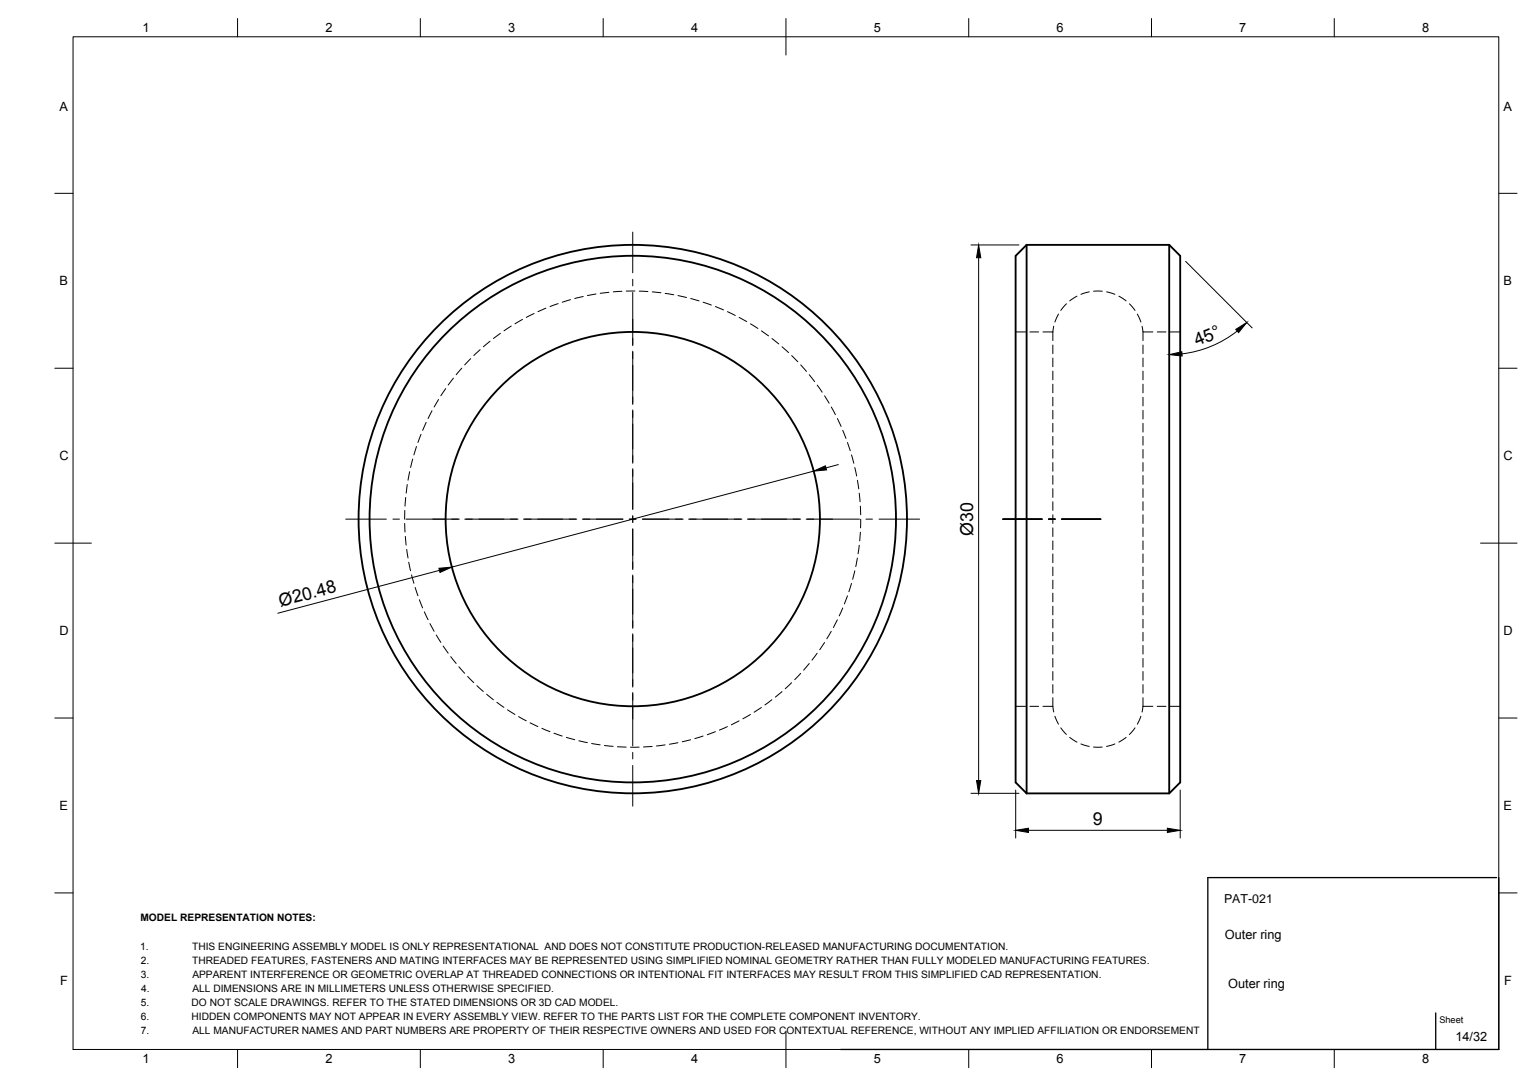
ISO-10303-21;
HEADER;
/* Generated by software containing ST-Developer
 * from STEP Tools, Inc. (www.steptools.com) 
 */

FILE_DESCRIPTION(
/* description */ ('Chain-less indexing wheel (Geneva) drive'),
/* implementation_level */ '2;1');

FILE_NAME(
/* name */ 'Outer ring.step',
/* time_stamp */ '2026-10-28T03:25:22-07:00',
/* author */ (''),
/* organization */ (''),
/* preprocessor_version */ 'ST-DEVELOPER v20.2',
/* originating_system */ 'Autodesk Translation Framework v15.17.0.0',
/* authorisation */ '');

FILE_SCHEMA (('AUTOMOTIVE_DESIGN { 1 0 10303 214 3 1 1 }'));
ENDSEC;

DATA;
#10=MECHANICAL_DESIGN_GEOMETRIC_PRESENTATION_REPRESENTATION('',(#311),#10957);
#196=TOROIDAL_SURFACE('',#6292,1.,0.247676);
#205=CONICAL_SURFACE('',#6303,1.47,0.785398163397449);
#206=CONICAL_SURFACE('',#6307,1.47,0.785398163397449);
#261=SHAPE_REPRESENTATION_RELATIONSHIP('SRR','None',#11075,#286);
#286=ADVANCED_BREP_SHAPE_REPRESENTATION('',(#343),#10938);
#311=STYLED_ITEM('',(#11287),#343);
#343=MANIFOLD_SOLID_BREP('Body1',#5708);
#426=FACE_BOUND('',#1180,.T.);
#427=FACE_BOUND('',#1185,.T.);
#541=PLANE('',#6300);
#542=PLANE('',#6309);
#785=FACE_OUTER_BOUND('',#1177,.T.);
#786=FACE_OUTER_BOUND('',#1178,.T.);
#787=FACE_OUTER_BOUND('',#1179,.T.);
#788=FACE_OUTER_BOUND('',#1181,.T.);
#789=FACE_OUTER_BOUND('',#1182,.T.);
#790=FACE_OUTER_BOUND('',#1183,.T.);
#791=FACE_OUTER_BOUND('',#1184,.T.);
#792=FACE_OUTER_BOUND('',#1186,.T.);
#1177=EDGE_LOOP('',(#4331,#4332,#4333,#4334,#4335,#4336));
#1178=EDGE_LOOP('',(#4337,#4338,#4339,#4340,#4341));
#1179=EDGE_LOOP('',(#4342));
#1180=EDGE_LOOP('',(#4343));
#1181=EDGE_LOOP('',(#4344,#4345,#4346,#4347));
#1182=EDGE_LOOP('',(#4348,#4349,#4350,#4351));
#1183=EDGE_LOOP('',(#4352,#4353,#4354,#4355));
#1184=EDGE_LOOP('',(#4356));
#1185=EDGE_LOOP('',(#4357));
#1186=EDGE_LOOP('',(#4358,#4359,#4360,#4361,#4362));
#1576=LINE('',#9299,#1950);
#1577=LINE('',#9308,#1951);
#1578=LINE('',#9312,#1952);
#1579=LINE('',#9316,#1953);
#1580=LINE('',#9319,#1954);
#1950=VECTOR('',#7482,1.023815);
#1951=VECTOR('',#7493,1.47);
#1952=VECTOR('',#7498,1.5);
#1953=VECTOR('',#7503,1.47);
#1954=VECTOR('',#7508,1.023815);
#2308=CIRCLE('',#6293,1.023815);
#2309=CIRCLE('',#6294,1.023815);
#2310=CIRCLE('',#6295,0.247676);
#2311=CIRCLE('',#6296,1.023815);
#2312=CIRCLE('',#6297,1.023815);
#2313=CIRCLE('',#6299,1.023815);
#2314=CIRCLE('',#6301,1.44);
#2315=CIRCLE('',#6302,1.023815);
#2316=CIRCLE('',#6304,1.5);
#2317=CIRCLE('',#6306,1.5);
#2318=CIRCLE('',#6308,1.44);
#2687=VERTEX_POINT('',#9287);
#2688=VERTEX_POINT('',#9288);
#2689=VERTEX_POINT('',#9291);
#2690=VERTEX_POINT('',#9293);
#2691=VERTEX_POINT('',#9297);
#2692=VERTEX_POINT('',#9301);
#2693=VERTEX_POINT('',#9303);
#2694=VERTEX_POINT('',#9306);
#2695=VERTEX_POINT('',#9310);
#2696=VERTEX_POINT('',#9314);
#3291=EDGE_CURVE('',#2687,#2688,#2308,.T.);
#3292=EDGE_CURVE('',#2688,#2687,#2309,.T.);
#3293=EDGE_CURVE('',#2688,#2689,#2310,.T.);
#3294=EDGE_CURVE('',#2690,#2689,#2311,.T.);
#3295=EDGE_CURVE('',#2689,#2690,#2312,.T.);
#3296=EDGE_CURVE('',#2691,#2691,#2313,.T.);
#3297=EDGE_CURVE('',#2691,#2690,#1576,.T.);
#3298=EDGE_CURVE('',#2692,#2692,#2314,.T.);
#3299=EDGE_CURVE('',#2693,#2693,#2315,.T.);
#3300=EDGE_CURVE('',#2694,#2694,#2316,.T.);
#3301=EDGE_CURVE('',#2694,#2692,#1577,.T.);
#3302=EDGE_CURVE('',#2695,#2695,#2317,.T.);
#3303=EDGE_CURVE('',#2695,#2694,#1578,.T.);
#3304=EDGE_CURVE('',#2696,#2696,#2318,.T.);
#3305=EDGE_CURVE('',#2696,#2695,#1579,.T.);
#3306=EDGE_CURVE('',#2687,#2693,#1580,.T.);
#4331=ORIENTED_EDGE('',*,*,#3291,.F.);
#4332=ORIENTED_EDGE('',*,*,#3292,.F.);
#4333=ORIENTED_EDGE('',*,*,#3293,.T.);
#4334=ORIENTED_EDGE('',*,*,#3294,.F.);
#4335=ORIENTED_EDGE('',*,*,#3295,.F.);
#4336=ORIENTED_EDGE('',*,*,#3293,.F.);
#4337=ORIENTED_EDGE('',*,*,#3296,.T.);
#4338=ORIENTED_EDGE('',*,*,#3297,.T.);
#4339=ORIENTED_EDGE('',*,*,#3294,.T.);
#4340=ORIENTED_EDGE('',*,*,#3295,.T.);
#4341=ORIENTED_EDGE('',*,*,#3297,.F.);
#4342=ORIENTED_EDGE('',*,*,#3298,.F.);
#4343=ORIENTED_EDGE('',*,*,#3299,.T.);
#4344=ORIENTED_EDGE('',*,*,#3300,.F.);
#4345=ORIENTED_EDGE('',*,*,#3301,.T.);
#4346=ORIENTED_EDGE('',*,*,#3298,.T.);
#4347=ORIENTED_EDGE('',*,*,#3301,.F.);
#4348=ORIENTED_EDGE('',*,*,#3302,.F.);
#4349=ORIENTED_EDGE('',*,*,#3303,.T.);
#4350=ORIENTED_EDGE('',*,*,#3300,.T.);
#4351=ORIENTED_EDGE('',*,*,#3303,.F.);
#4352=ORIENTED_EDGE('',*,*,#3304,.F.);
#4353=ORIENTED_EDGE('',*,*,#3305,.T.);
#4354=ORIENTED_EDGE('',*,*,#3302,.T.);
#4355=ORIENTED_EDGE('',*,*,#3305,.F.);
#4356=ORIENTED_EDGE('',*,*,#3304,.T.);
#4357=ORIENTED_EDGE('',*,*,#3296,.F.);
#4358=ORIENTED_EDGE('',*,*,#3291,.T.);
#4359=ORIENTED_EDGE('',*,*,#3292,.T.);
#4360=ORIENTED_EDGE('',*,*,#3306,.T.);
#4361=ORIENTED_EDGE('',*,*,#3299,.F.);
#4362=ORIENTED_EDGE('',*,*,#3306,.F.);
#5300=CYLINDRICAL_SURFACE('',#6298,1.023815);
#5301=CYLINDRICAL_SURFACE('',#6305,1.5);
#5302=CYLINDRICAL_SURFACE('',#6310,1.023815);
#5499=ADVANCED_FACE('',(#785),#196,.F.);
#5500=ADVANCED_FACE('',(#786),#5300,.F.);
#5501=ADVANCED_FACE('',(#787,#426),#541,.T.);
#5502=ADVANCED_FACE('',(#788),#205,.T.);
#5503=ADVANCED_FACE('',(#789),#5301,.T.);
#5504=ADVANCED_FACE('',(#790),#206,.T.);
#5505=ADVANCED_FACE('',(#791,#427),#542,.T.);
#5506=ADVANCED_FACE('',(#792),#5302,.F.);
#5708=CLOSED_SHELL('',(#5499,#5500,#5501,#5502,#5503,#5504,#5505,#5506));
#6291=AXIS2_PLACEMENT_3D('',#9285,#7464,#7465);
#6292=AXIS2_PLACEMENT_3D('',#9286,#7466,#7467);
#6293=AXIS2_PLACEMENT_3D('',#9289,#7468,#7469);
#6294=AXIS2_PLACEMENT_3D('',#9290,#7470,#7471);
#6295=AXIS2_PLACEMENT_3D('',#9292,#7472,#7473);
#6296=AXIS2_PLACEMENT_3D('',#9294,#7474,#7475);
#6297=AXIS2_PLACEMENT_3D('',#9295,#7476,#7477);
#6298=AXIS2_PLACEMENT_3D('',#9296,#7478,#7479);
#6299=AXIS2_PLACEMENT_3D('',#9298,#7480,#7481);
#6300=AXIS2_PLACEMENT_3D('',#9300,#7483,#7484);
#6301=AXIS2_PLACEMENT_3D('',#9302,#7485,#7486);
#6302=AXIS2_PLACEMENT_3D('',#9304,#7487,#7488);
#6303=AXIS2_PLACEMENT_3D('',#9305,#7489,#7490);
#6304=AXIS2_PLACEMENT_3D('',#9307,#7491,#7492);
#6305=AXIS2_PLACEMENT_3D('',#9309,#7494,#7495);
#6306=AXIS2_PLACEMENT_3D('',#9311,#7496,#7497);
#6307=AXIS2_PLACEMENT_3D('',#9313,#7499,#7500);
#6308=AXIS2_PLACEMENT_3D('',#9315,#7501,#7502);
#6309=AXIS2_PLACEMENT_3D('',#9317,#7504,#7505);
#6310=AXIS2_PLACEMENT_3D('',#9318,#7506,#7507);
#7464=DIRECTION('axis',(0.,0.,1.));
#7465=DIRECTION('refdir',(1.,0.,0.));
#7466=DIRECTION('center_axis',(0.,-1.,0.));
#7467=DIRECTION('ref_axis',(0.,0.,-1.));
#7468=DIRECTION('center_axis',(0.,-1.,0.));
#7469=DIRECTION('ref_axis',(1.,0.,0.));
#7470=DIRECTION('center_axis',(0.,-1.,0.));
#7471=DIRECTION('ref_axis',(1.,0.,0.));
#7472=DIRECTION('center_axis',(1.,0.,1.22464679914735E-16));
#7473=DIRECTION('ref_axis',(-1.22464679914735E-16,0.,1.));
#7474=DIRECTION('center_axis',(0.,1.,0.));
#7475=DIRECTION('ref_axis',(1.,0.,0.));
#7476=DIRECTION('center_axis',(0.,1.,0.));
#7477=DIRECTION('ref_axis',(1.,0.,0.));
#7478=DIRECTION('center_axis',(0.,-1.,0.));
#7479=DIRECTION('ref_axis',(1.,0.,0.));
#7480=DIRECTION('center_axis',(0.,-1.,0.));
#7481=DIRECTION('ref_axis',(1.,0.,0.));
#7482=DIRECTION('',(0.,1.,0.));
#7483=DIRECTION('center_axis',(0.,1.,0.));
#7484=DIRECTION('ref_axis',(0.,0.,1.));
#7485=DIRECTION('center_axis',(0.,-1.,0.));
#7486=DIRECTION('ref_axis',(1.,0.,0.));
#7487=DIRECTION('center_axis',(0.,-1.,0.));
#7488=DIRECTION('ref_axis',(1.,0.,0.));
#7489=DIRECTION('center_axis',(0.,-1.,0.));
#7490=DIRECTION('ref_axis',(1.,0.,0.));
#7491=DIRECTION('center_axis',(0.,-1.,0.));
#7492=DIRECTION('ref_axis',(1.,0.,0.));
#7493=DIRECTION('',(0.707106781186548,0.707106781186547,8.65956056235494E-17));
#7494=DIRECTION('center_axis',(0.,-1.,0.));
#7495=DIRECTION('ref_axis',(1.,0.,0.));
#7496=DIRECTION('center_axis',(0.,-1.,0.));
#7497=DIRECTION('ref_axis',(1.,0.,0.));
#7498=DIRECTION('',(0.,1.,0.));
#7499=DIRECTION('center_axis',(0.,1.,0.));
#7500=DIRECTION('ref_axis',(1.,0.,0.));
#7501=DIRECTION('center_axis',(0.,-1.,0.));
#7502=DIRECTION('ref_axis',(1.,0.,0.));
#7503=DIRECTION('',(-0.707106781186548,0.707106781186547,-8.65956056235494E-17));
#7504=DIRECTION('center_axis',(0.,-1.,0.));
#7505=DIRECTION('ref_axis',(0.,0.,-1.));
#7506=DIRECTION('center_axis',(0.,-1.,0.));
#7507=DIRECTION('ref_axis',(1.,0.,0.));
#7508=DIRECTION('',(0.,1.,0.));
#9285=CARTESIAN_POINT('',(0.,0.,0.));
#9286=CARTESIAN_POINT('Origin',(0.,0.,0.));
#9287=CARTESIAN_POINT('',(-1.023815,0.246528389340863,-1.25381176266905E-16));
#9288=CARTESIAN_POINT('',(-1.25381176266905E-16,0.246528389340863,1.023815));
#9289=CARTESIAN_POINT('Origin',(0.,0.246528389340863,0.));
#9290=CARTESIAN_POINT('Origin',(0.,0.246528389340863,0.));
#9291=CARTESIAN_POINT('',(-1.25381176266905E-16,-0.246528389340863,1.023815));
#9292=CARTESIAN_POINT('Origin',(-1.22464679914735E-16,0.,1.));
#9293=CARTESIAN_POINT('',(-1.023815,-0.246528389340863,1.25381176266905E-16));
#9294=CARTESIAN_POINT('Origin',(0.,-0.246528389340863,0.));
#9295=CARTESIAN_POINT('Origin',(0.,-0.246528389340863,0.));
#9296=CARTESIAN_POINT('Origin',(0.,0.,0.));
#9297=CARTESIAN_POINT('',(-1.023815,-0.45,-1.25381176266905E-16));
#9298=CARTESIAN_POINT('Origin',(0.,-0.45,0.));
#9299=CARTESIAN_POINT('',(-1.023815,0.,-1.25381176266905E-16));
#9300=CARTESIAN_POINT('Origin',(1.44,0.45,0.));
#9301=CARTESIAN_POINT('',(-1.44,0.45,-1.76349139077219E-16));
#9302=CARTESIAN_POINT('Origin',(0.,0.45,0.));
#9303=CARTESIAN_POINT('',(-1.023815,0.45,-1.25381176266905E-16));
#9304=CARTESIAN_POINT('Origin',(0.,0.45,0.));
#9305=CARTESIAN_POINT('Origin',(0.,0.42,0.));
#9306=CARTESIAN_POINT('',(-1.5,0.39,-1.83697019872103E-16));
#9307=CARTESIAN_POINT('Origin',(0.,0.39,0.));
#9308=CARTESIAN_POINT('',(-1.47,0.42,-1.80023079474661E-16));
#9309=CARTESIAN_POINT('Origin',(0.,0.,0.));
#9310=CARTESIAN_POINT('',(-1.5,-0.39,-1.83697019872103E-16));
#9311=CARTESIAN_POINT('Origin',(0.,-0.39,0.));
#9312=CARTESIAN_POINT('',(-1.5,0.,-1.83697019872103E-16));
#9313=CARTESIAN_POINT('Origin',(0.,-0.42,0.));
#9314=CARTESIAN_POINT('',(-1.44,-0.45,-1.76349139077219E-16));
#9315=CARTESIAN_POINT('Origin',(0.,-0.45,0.));
#9316=CARTESIAN_POINT('',(-1.47,-0.42,-1.80023079474661E-16));
#9317=CARTESIAN_POINT('Origin',(1.023815,-0.45,0.));
#9318=CARTESIAN_POINT('Origin',(0.,0.,0.));
#9319=CARTESIAN_POINT('',(-1.023815,0.,-1.25381176266905E-16));
#10907=UNCERTAINTY_MEASURE_WITH_UNIT(LENGTH_MEASURE(0.001),#10958,
'DISTANCE_ACCURACY_VALUE',
'Maximum model space distance between geometric entities at asserted c
onnectivities');
#10926=UNCERTAINTY_MEASURE_WITH_UNIT(LENGTH_MEASURE(0.001),#10958,
'DISTANCE_ACCURACY_VALUE',
'Maximum model space distance between geometric entities at asserted c
onnectivities');
#10938=(
GEOMETRIC_REPRESENTATION_CONTEXT(3)
GLOBAL_UNCERTAINTY_ASSIGNED_CONTEXT((#10907))
GLOBAL_UNIT_ASSIGNED_CONTEXT((#10958,#10960,#10961))
REPRESENTATION_CONTEXT('','3D')
);
#10957=(
GEOMETRIC_REPRESENTATION_CONTEXT(3)
GLOBAL_UNCERTAINTY_ASSIGNED_CONTEXT((#10926))
GLOBAL_UNIT_ASSIGNED_CONTEXT((#10958,#10960,#10961))
REPRESENTATION_CONTEXT('','3D')
);
#10958=(
LENGTH_UNIT()
NAMED_UNIT(*)
SI_UNIT(.CENTI.,.METRE.)
);
#10960=(
NAMED_UNIT(*)
PLANE_ANGLE_UNIT()
SI_UNIT($,.RADIAN.)
);
#10961=(
NAMED_UNIT(*)
SI_UNIT($,.STERADIAN.)
SOLID_ANGLE_UNIT()
);
#10973=SHAPE_DEFINITION_REPRESENTATION(#11003,#11075);
#11003=PRODUCT_DEFINITION_SHAPE('',$,#11106);
#11075=SHAPE_REPRESENTATION('',(#6291),#10938);
#11094=PRODUCT_DEFINITION_CONTEXT('part definition',#11186,'design');
#11106=PRODUCT_DEFINITION('Outer ring','Outer ring',#11136,#11094);
#11136=PRODUCT_DEFINITION_FORMATION('',$,#11199);
#11186=APPLICATION_CONTEXT(
'Core Data for Automotive Mechanical Design Process');
#11187=PRODUCT_CONTEXT('part definition',#11186,'mechanical');
#11199=PRODUCT('Outer ring','Outer ring','Outer ring',(#11187));
#11281=COLOUR_RGB('Grey',0.48,0.52,0.57);
#11282=FILL_AREA_STYLE_COLOUR('',#11281);
#11283=FILL_AREA_STYLE('',(#11282));
#11284=SURFACE_STYLE_FILL_AREA(#11283);
#11285=SURFACE_SIDE_STYLE('',(#11284));
#11286=SURFACE_STYLE_USAGE(.BOTH.,#11285);
#11287=PRESENTATION_STYLE_ASSIGNMENT((#11286));
ENDSEC;
END-ISO-10303-21;
